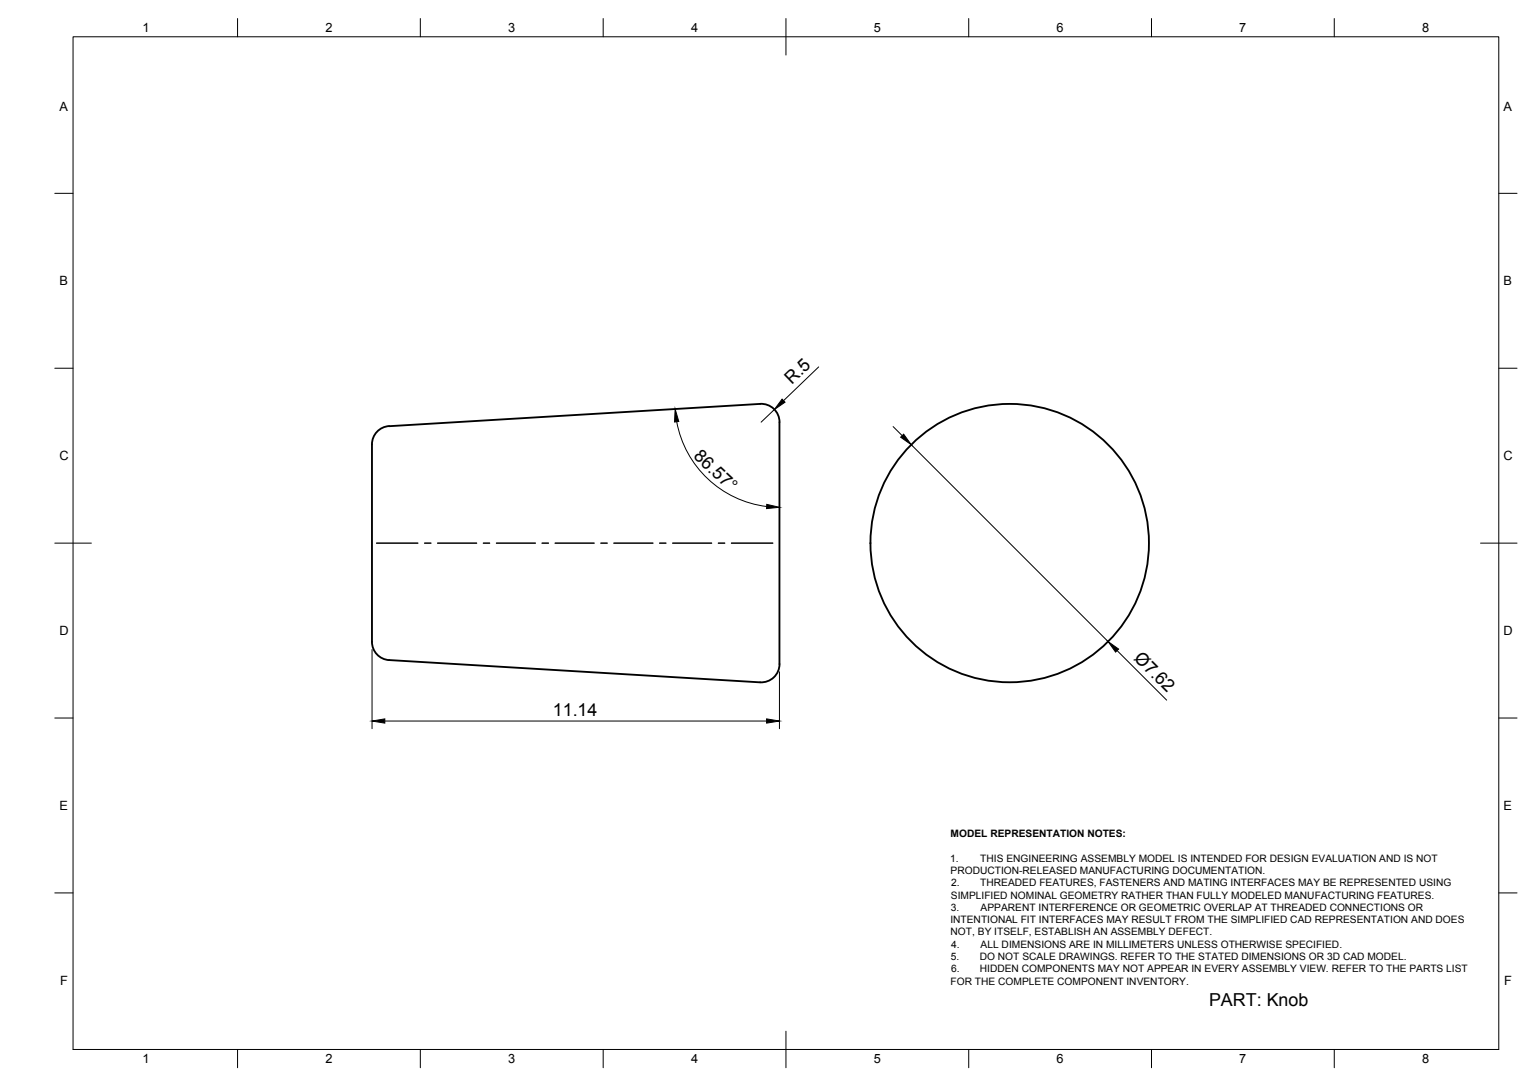
ISO-10303-21;
HEADER;
/* Generated by software containing ST-Developer
 * from STEP Tools, Inc. (www.steptools.com) 
 */

FILE_DESCRIPTION(
/* description */ (''),
/* implementation_level */ '2;1');

FILE_NAME(
/* name */ 'Knob.step',
/* time_stamp */ '2026-10-05T01:33:24-07:00',
/* author */ (''),
/* organization */ (''),
/* preprocessor_version */ 'ST-DEVELOPER v20.2',
/* originating_system */ 'Autodesk Translation Framework v15.15.0.0',
/* authorisation */ '');

FILE_SCHEMA (('AUTOMOTIVE_DESIGN { 1 0 10303 214 3 1 1 }'));
ENDSEC;

DATA;
#10=MECHANICAL_DESIGN_GEOMETRIC_PRESENTATION_REPRESENTATION('',(#85),#1128);
#52=TOROIDAL_SURFACE('',#673,3.3075988470339,0.49999999999999);
#53=TOROIDAL_SURFACE('',#678,2.69979677377649,0.500000000000025);
#57=CONICAL_SURFACE('',#676,3.50280261490539,0.0598485673150425);
#65=SHAPE_REPRESENTATION_RELATIONSHIP('SRR','None',#1169,#75);
#75=ADVANCED_BREP_SHAPE_REPRESENTATION('',(#95),#1121);
#85=STYLED_ITEM('',(#1225),#95);
#95=MANIFOLD_SOLID_BREP('Body1',#524);
#108=LINE('',#1010,#125);
#125=VECTOR('',#817,3.50280261490539);
#159=FACE_OUTER_BOUND('',#200,.T.);
#160=FACE_OUTER_BOUND('',#201,.T.);
#161=FACE_OUTER_BOUND('',#202,.T.);
#162=FACE_OUTER_BOUND('',#203,.T.);
#163=FACE_OUTER_BOUND('',#204,.T.);
#200=EDGE_LOOP('',(#386));
#201=EDGE_LOOP('',(#387,#388,#389,#390));
#202=EDGE_LOOP('',(#391,#392,#393,#394));
#203=EDGE_LOOP('',(#395,#396,#397,#398));
#204=EDGE_LOOP('',(#399));
#239=CIRCLE('',#672,3.3075988470339);
#240=CIRCLE('',#674,3.80670365153407);
#241=CIRCLE('',#675,0.49999999999999);
#242=CIRCLE('',#677,3.1989015782767);
#243=CIRCLE('',#679,2.69979677377651);
#244=CIRCLE('',#680,0.500000000000025);
#275=VERTEX_POINT('',#1002);
#276=VERTEX_POINT('',#1005);
#277=VERTEX_POINT('',#1009);
#278=VERTEX_POINT('',#1013);
#315=EDGE_CURVE('',#275,#275,#239,.T.);
#316=EDGE_CURVE('',#276,#276,#240,.T.);
#317=EDGE_CURVE('',#276,#275,#241,.T.);
#318=EDGE_CURVE('',#276,#277,#108,.T.);
#319=EDGE_CURVE('',#277,#277,#242,.T.);
#320=EDGE_CURVE('',#278,#278,#243,.T.);
#321=EDGE_CURVE('',#278,#277,#244,.T.);
#386=ORIENTED_EDGE('',*,*,#315,.F.);
#387=ORIENTED_EDGE('',*,*,#316,.F.);
#388=ORIENTED_EDGE('',*,*,#317,.T.);
#389=ORIENTED_EDGE('',*,*,#315,.T.);
#390=ORIENTED_EDGE('',*,*,#317,.F.);
#391=ORIENTED_EDGE('',*,*,#316,.T.);
#392=ORIENTED_EDGE('',*,*,#318,.T.);
#393=ORIENTED_EDGE('',*,*,#319,.F.);
#394=ORIENTED_EDGE('',*,*,#318,.F.);
#395=ORIENTED_EDGE('',*,*,#320,.F.);
#396=ORIENTED_EDGE('',*,*,#321,.T.);
#397=ORIENTED_EDGE('',*,*,#319,.T.);
#398=ORIENTED_EDGE('',*,*,#321,.F.);
#399=ORIENTED_EDGE('',*,*,#320,.T.);
#466=PLANE('',#671);
#467=PLANE('',#681);
#493=ADVANCED_FACE('',(#159),#466,.T.);
#494=ADVANCED_FACE('',(#160),#52,.T.);
#495=ADVANCED_FACE('',(#161),#57,.T.);
#496=ADVANCED_FACE('',(#162),#53,.T.);
#497=ADVANCED_FACE('',(#163),#467,.T.);
#524=CLOSED_SHELL('',(#493,#494,#495,#496,#497));
#670=AXIS2_PLACEMENT_3D('',#1000,#803,#804);
#671=AXIS2_PLACEMENT_3D('',#1001,#805,#806);
#672=AXIS2_PLACEMENT_3D('',#1003,#807,#808);
#673=AXIS2_PLACEMENT_3D('',#1004,#809,#810);
#674=AXIS2_PLACEMENT_3D('',#1006,#811,#812);
#675=AXIS2_PLACEMENT_3D('',#1007,#813,#814);
#676=AXIS2_PLACEMENT_3D('',#1008,#815,#816);
#677=AXIS2_PLACEMENT_3D('',#1011,#818,#819);
#678=AXIS2_PLACEMENT_3D('',#1012,#820,#821);
#679=AXIS2_PLACEMENT_3D('',#1014,#822,#823);
#680=AXIS2_PLACEMENT_3D('',#1015,#824,#825);
#681=AXIS2_PLACEMENT_3D('',#1016,#826,#827);
#803=DIRECTION('axis',(0.,0.,1.));
#804=DIRECTION('refdir',(1.,0.,0.));
#805=DIRECTION('center_axis',(-1.,0.,0.));
#806=DIRECTION('ref_axis',(0.,0.,1.));
#807=DIRECTION('center_axis',(1.,0.,0.));
#808=DIRECTION('ref_axis',(0.,0.,-1.));
#809=DIRECTION('center_axis',(1.,0.,0.));
#810=DIRECTION('ref_axis',(0.,0.,-1.));
#811=DIRECTION('center_axis',(1.,0.,0.));
#812=DIRECTION('ref_axis',(0.,0.,-1.));
#813=DIRECTION('center_axis',(0.,-1.,-1.22464679914735E-16));
#814=DIRECTION('ref_axis',(0.,-1.22464679914735E-16,1.));
#815=DIRECTION('center_axis',(-1.,0.,0.));
#816=DIRECTION('ref_axis',(0.,0.,-1.));
#817=DIRECTION('',(0.998209609000375,-7.32496099175571E-18,-0.0598128456045909));
#818=DIRECTION('center_axis',(1.,0.,0.));
#819=DIRECTION('ref_axis',(0.,0.,-1.));
#820=DIRECTION('center_axis',(1.,0.,0.));
#821=DIRECTION('ref_axis',(0.,0.,-1.));
#822=DIRECTION('center_axis',(1.,0.,0.));
#823=DIRECTION('ref_axis',(0.,0.,-1.));
#824=DIRECTION('center_axis',(0.,-1.,-1.22464679914735E-16));
#825=DIRECTION('ref_axis',(0.,-1.22464679914735E-16,1.));
#826=DIRECTION('center_axis',(1.,0.,0.));
#827=DIRECTION('ref_axis',(0.,0.,-1.));
#1000=CARTESIAN_POINT('',(0.,0.,0.));
#1001=CARTESIAN_POINT('Origin',(88.8564620398316,0.,-3.3075988470339));
#1002=CARTESIAN_POINT('',(88.8564620398316,-4.05064034088354E-16,3.3075988470339));
#1003=CARTESIAN_POINT('Origin',(88.8564620398316,0.,0.));
#1004=CARTESIAN_POINT('Origin',(89.3564620398316,0.,0.));
#1005=CARTESIAN_POINT('',(89.3863684626339,-4.66186744215375E-16,3.80670365153407));
#1006=CARTESIAN_POINT('Origin',(89.3863684626339,0.,0.));
#1007=CARTESIAN_POINT('Origin',(89.3564620398316,-4.05064034088354E-16,
3.3075988470339));
#1008=CARTESIAN_POINT('Origin',(94.4581374427181,0.,0.));
#1009=CARTESIAN_POINT('',(99.5299064228023,-3.91752457862398E-16,3.1989015782767));
#1010=CARTESIAN_POINT('',(94.4581374427181,4.28969601038887E-16,3.50280261490539));
#1011=CARTESIAN_POINT('Origin',(99.5299064228023,0.,0.));
#1012=CARTESIAN_POINT('Origin',(99.5,0.,0.));
#1013=CARTESIAN_POINT('',(100.,-3.30629747735376E-16,2.69979677377651));
#1014=CARTESIAN_POINT('Origin',(100.,0.,0.));
#1015=CARTESIAN_POINT('Origin',(99.5,-3.30629747735373E-16,2.69979677377649));
#1016=CARTESIAN_POINT('Origin',(100.,0.,0.));
#1109=UNCERTAINTY_MEASURE_WITH_UNIT(LENGTH_MEASURE(0.01),#1129,
'DISTANCE_ACCURACY_VALUE',
'Maximum model space distance between geometric entities at asserted c
onnectivities');
#1116=UNCERTAINTY_MEASURE_WITH_UNIT(LENGTH_MEASURE(0.01),#1129,
'DISTANCE_ACCURACY_VALUE',
'Maximum model space distance between geometric entities at asserted c
onnectivities');
#1121=(
GEOMETRIC_REPRESENTATION_CONTEXT(3)
GLOBAL_UNCERTAINTY_ASSIGNED_CONTEXT((#1109))
GLOBAL_UNIT_ASSIGNED_CONTEXT((#1129,#1131,#1132))
REPRESENTATION_CONTEXT('','3D')
);
#1128=(
GEOMETRIC_REPRESENTATION_CONTEXT(3)
GLOBAL_UNCERTAINTY_ASSIGNED_CONTEXT((#1116))
GLOBAL_UNIT_ASSIGNED_CONTEXT((#1129,#1131,#1132))
REPRESENTATION_CONTEXT('','3D')
);
#1129=(
LENGTH_UNIT()
NAMED_UNIT(*)
SI_UNIT(.MILLI.,.METRE.)
);
#1131=(
NAMED_UNIT(*)
PLANE_ANGLE_UNIT()
SI_UNIT($,.RADIAN.)
);
#1132=(
NAMED_UNIT(*)
SI_UNIT($,.STERADIAN.)
SOLID_ANGLE_UNIT()
);
#1137=SHAPE_DEFINITION_REPRESENTATION(#1148,#1169);
#1148=PRODUCT_DEFINITION_SHAPE('',$,#1181);
#1169=SHAPE_REPRESENTATION('',(#670),#1121);
#1176=PRODUCT_DEFINITION_CONTEXT('part definition',#1211,'design');
#1181=PRODUCT_DEFINITION('Knob','Knob',#1192,#1176);
#1192=PRODUCT_DEFINITION_FORMATION('',$,#1217);
#1211=APPLICATION_CONTEXT(
'Core Data for Automotive Mechanical Design Process');
#1212=PRODUCT_CONTEXT('part definition',#1211,'mechanical');
#1217=PRODUCT('Knob','Knob',$,(#1212));
#1225=PRESENTATION_STYLE_ASSIGNMENT((#1229));
#1229=SURFACE_STYLE_USAGE(.BOTH.,#1233);
#1233=SURFACE_SIDE_STYLE('',(#1237));
#1237=SURFACE_STYLE_FILL_AREA(#1241);
#1241=FILL_AREA_STYLE('Opaque(201,201,201)',(#1245));
#1245=FILL_AREA_STYLE_COLOUR('Opaque(201,201,201)',#1249);
#1249=COLOUR_RGB('Opaque(201,201,201)', 0.09019608, 0.27058824, 0.51372549);
ENDSEC;
END-ISO-10303-21;
